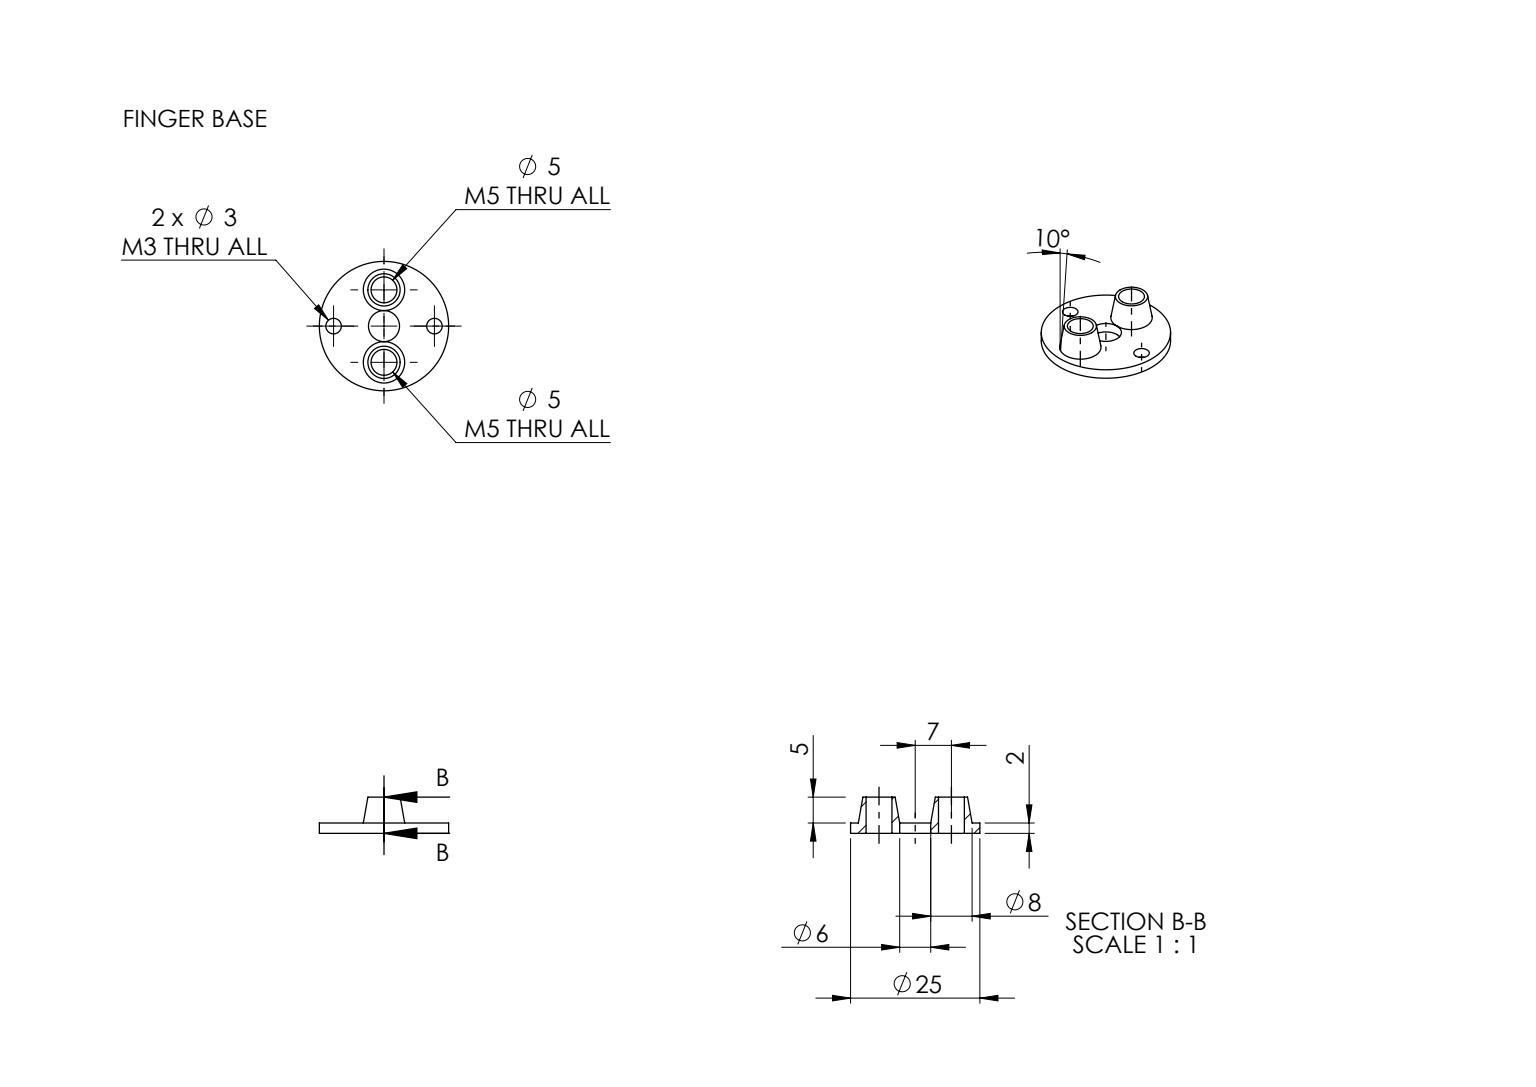
ISO-10303-21;
HEADER;
FILE_DESCRIPTION (('STEP AP214'),
    '1' );
FILE_NAME ('finger base.step',
    '2026-10-04T10:31:01',
    ( '' ),
    ( '' ),
    'SwSTEP 2.0',
    'SolidWorks 2026',
    '' );
FILE_SCHEMA (( 'AUTOMOTIVE_DESIGN' ));
ENDSEC;

DATA;
#8=ORIENTED_EDGE ( 'NONE', *, *, #4476, .T. ) ;
#18=LINE ( 'NONE', #14576, #2348 ) ;
#22=CARTESIAN_POINT ( 'NONE',  ( -3.061616997868391523E-16, 189.0000000000000000, -7.000000000000000000 ) ) ;
#42=EDGE_CURVE ( 'NONE', #14222, #12950, #1605, .T. ) ;
#113=EDGE_CURVE ( 'NONE', #5247, #7816, #14877, .T. ) ;
#127=CARTESIAN_POINT ( 'NONE',  ( 0.000000000000000000, 184.0000000000000000, 0.000000000000000000 ) ) ;
#147=DIRECTION ( 'NONE',  ( -1.000000000000000000, 0.000000000000000000, 0.000000000000000000 ) ) ;
#166=PRODUCT ( 'finger base', 'finger base', '', ( #15382 ) ) ;
#182=DIRECTION ( 'NONE',  ( -0.1736481776669306920, -0.9848077530122080203, 0.000000000000000000 ) ) ;
#199=CIRCLE ( 'NONE', #5549, 2.499999999999999556 ) ;
#215=SURFACE_SIDE_STYLE ('',( #11110 ) ) ;
#260=VERTEX_POINT ( 'NONE', #5788 ) ;
#261=ORIENTED_EDGE ( 'NONE', *, *, #6781, .F. ) ;
#280=DIRECTION ( 'NONE',  ( -6.123233995736766036E-17, 1.000000000000000000, 0.000000000000000000 ) ) ;
#285=AXIS2_PLACEMENT_3D ( 'NONE', #127, #3629, #8659 ) ;
#315=ORIENTED_EDGE ( 'NONE', *, *, #1912, .F. ) ;
#323=SURFACE_STYLE_FILL_AREA ( #10269 ) ;
#424=AXIS2_PLACEMENT_3D ( 'NONE', #6276, #8742, #11195 ) ;
#466=CARTESIAN_POINT ( 'NONE',  ( 0.000000000000000000, 184.0000000000000000, 0.000000000000000000 ) ) ;
#476=DIRECTION ( 'NONE',  ( 0.000000000000000000, 0.000000000000000000, 1.000000000000000000 ) ) ;
#481=DIRECTION ( 'NONE',  ( -6.123233995736766036E-17, 1.000000000000000000, 0.000000000000000000 ) ) ;
#509=ORIENTED_EDGE ( 'NONE', *, *, #12250, .F. ) ;
#550=ADVANCED_FACE ( 'NONE', ( #2271 ), #7141, .T. ) ;
#552=DIRECTION ( 'NONE',  ( -6.123233995736766036E-17, 1.000000000000000000, 0.000000000000000000 ) ) ;
#561=DIRECTION ( 'NONE',  ( -0.000000000000000000, 1.000000000000000000, -0.000000000000000000 ) ) ;
#562=PLANE ( 'NONE',  #12276 ) ;
#622=ORIENTED_EDGE ( 'NONE', *, *, #10760, .T. ) ;
#633=DIRECTION ( 'NONE',  ( 0.000000000000000000, 0.000000000000000000, 1.000000000000000000 ) ) ;
#640=EDGE_LOOP ( 'NONE', ( #3910, #10945 ) ) ;
#650=CARTESIAN_POINT ( 'NONE',  ( -9.148167235839370302E-31, 189.0000000000000000, 4.500000000000000888 ) ) ;
#658=ORIENTED_EDGE ( 'NONE', *, *, #14770, .T. ) ;
#700=CONICAL_SURFACE ( 'NONE', #15707, 4.000000000000001776, 0.1745329251994333364 ) ;
#702=CIRCLE ( 'NONE', #11125, 12.49999999999999822 ) ;
#742=CIRCLE ( 'NONE', #2268, 1.499999999999999556 ) ;
#803=AXIS2_PLACEMENT_3D ( 'NONE', #2594, #12294, #1393 ) ;
#842=EDGE_CURVE ( 'NONE', #7816, #5381, #5978, .T. ) ;
#847=ORIENTED_EDGE ( 'NONE', *, *, #12750, .T. ) ;
#877=EDGE_CURVE ( 'NONE', #5381, #5666, #1680, .T. ) ;
#896=CARTESIAN_POINT ( 'NONE',  ( -4.000000000000002665, 184.0000000000000000, -7.000000000000000000 ) ) ;
#918=AXIS2_PLACEMENT_3D ( 'NONE', #466, #15034, #6295 ) ;
#934=DIRECTION ( 'NONE',  ( -6.123233995736766036E-17, 1.000000000000000000, 0.000000000000000000 ) ) ;
#955=DIRECTION ( 'NONE',  ( 1.000000000000000000, 6.123233995736766036E-17, 0.000000000000000000 ) ) ;
#990=CARTESIAN_POINT ( 'NONE',  ( 0.000000000000000000, 184.0000000000000000, 2.999999999999998224 ) ) ;
#999=AXIS2_PLACEMENT_3D ( 'NONE', #13899, #6603, #9146 ) ;
#1019=ORIENTED_EDGE ( 'NONE', *, *, #5618, .F. ) ;
#1037=ADVANCED_FACE ( 'NONE', ( #2861 ), #6531, .F. ) ;
#1043=EDGE_CURVE ( 'NONE', #4972, #8636, #4494, .T. ) ;
#1061=VERTEX_POINT ( 'NONE', #12635 ) ;
#1081=EDGE_LOOP ( 'NONE', ( #14981, #4075, #14585, #5983 ) ) ;
#1165=( NAMED_UNIT ( * ) PLANE_ANGLE_UNIT ( ) SI_UNIT ( $, .RADIAN. ) );
#1203=AXIS2_PLACEMENT_3D ( 'NONE', #11068, #5988, #10992 ) ;
#1257=ADVANCED_FACE ( 'NONE', ( #11272 ), #7034, .T. ) ;
#1260=CARTESIAN_POINT ( 'NONE',  ( 1.530808498934191324E-15, 184.0000000000000000, 12.49999999999999822 ) ) ;
#1347=CARTESIAN_POINT ( 'NONE',  ( 9.750000000000003553, 184.0000000000000000, 1.020968533498575461E-13 ) ) ;
#1355=EDGE_CURVE ( 'NONE', #5666, #5381, #15411, .T. ) ;
#1370=ORIENTED_EDGE ( 'NONE', *, *, #3477, .F. ) ;
#1388=CARTESIAN_POINT ( 'NONE',  ( -3.061616997868391523E-16, 182.0000000000000000, 7.000000000000000000 ) ) ;
#1393=DIRECTION ( 'NONE',  ( -1.000000000000000000, 0.000000000000000000, 0.000000000000000000 ) ) ;
#1418=VECTOR ( 'NONE', #14560, 1000.000000000000000 ) ;
#1427=ADVANCED_FACE ( 'NONE', ( #12848 ), #1951, .F. ) ;
#1463=VECTOR ( 'NONE', #561, 1000.000000000000000 ) ;
#1473=DIRECTION ( 'NONE',  ( 0.000000000000000000, 0.000000000000000000, 1.000000000000000000 ) ) ;
#1488=ORIENTED_EDGE ( 'NONE', *, *, #10760, .F. ) ;
#1491=CARTESIAN_POINT ( 'NONE',  ( -3.061616997868386099E-16, 189.0000000000000000, 7.000000000000000000 ) ) ;
#1589=FILL_AREA_STYLE_COLOUR ( '', #14448 ) ;
#1605=LINE ( 'NONE', #2653, #14618 ) ;
#1609=CONICAL_SURFACE ( 'NONE', #3645, 4.000000000000002665, 0.1745329251994333364 ) ;
#1651=DIRECTION ( 'NONE',  ( 1.000000000000000000, 0.000000000000000000, 0.000000000000000000 ) ) ;
#1658=DIRECTION ( 'NONE',  ( -0.000000000000000000, 1.000000000000000000, -0.000000000000000000 ) ) ;
#1679=EDGE_LOOP ( 'NONE', ( #2885, #13212 ) ) ;
#1680=CIRCLE ( 'NONE', #12608, 1.499999999999999556 ) ;
#1701=CARTESIAN_POINT ( 'NONE',  ( 3.118365096457674568, 189.0000000000000000, -7.000000000000000888 ) ) ;
#1715=CARTESIAN_POINT ( 'NONE',  ( -9.750000000000003553, 184.0000000000000000, -3.401296724241641415E-14 ) ) ;
#1721=AXIS2_PLACEMENT_3D ( 'NONE', #13992, #15511, #9156 ) ;
#1725=VECTOR ( 'NONE', #7804, 1000.000000000000000 ) ;
#1726=DIRECTION ( 'NONE',  ( -6.123233995736766036E-17, 1.000000000000000000, 0.000000000000000000 ) ) ;
#1736=AXIS2_PLACEMENT_3D ( 'NONE', #2792, #8928, #476 ) ;
#1743=CYLINDRICAL_SURFACE ( 'NONE', #1746, 2.499999999999999556 ) ;
#1746=AXIS2_PLACEMENT_3D ( 'NONE', #5265, #10342, #12567 ) ;
#1809=CARTESIAN_POINT ( 'NONE',  ( -3.061616997868391523E-16, 189.0000000000000000, -7.000000000000000000 ) ) ;
#1833=ORIENTED_EDGE ( 'NONE', *, *, #2892, .T. ) ;
#1898=DIRECTION ( 'NONE',  ( -1.000000000000000000, 0.000000000000000000, 0.000000000000000000 ) ) ;
#1908=AXIS2_PLACEMENT_3D ( 'NONE', #3067, #5542, #5467 ) ;
#1912=EDGE_CURVE ( 'NONE', #2813, #6711, #6038, .T. ) ;
#1931=CYLINDRICAL_SURFACE ( 'NONE', #4961, 1.499999999999999556 ) ;
#1951=CYLINDRICAL_SURFACE ( 'NONE', #5267, 1.499999999999999556 ) ;
#1981=DIRECTION ( 'NONE',  ( 0.000000000000000000, 0.000000000000000000, 1.000000000000000000 ) ) ;
#1997=CARTESIAN_POINT ( 'NONE',  ( 9.750000000000003553, 184.0000000000000000, 1.020968533498575461E-13 ) ) ;
#2021=CYLINDRICAL_SURFACE ( 'NONE', #1908, 12.49999999999999822 ) ;
#2054=VERTEX_POINT ( 'NONE', #13437 ) ;
#2057=CYLINDRICAL_SURFACE ( 'NONE', #5024, 2.499999999999999556 ) ;
#2067=FACE_BOUND ( 'NONE', #14789, .T. ) ;
#2071=AXIS2_PLACEMENT_3D ( 'NONE', #15163, #5148, #1473 ) ;
#2095=ORIENTED_EDGE ( 'NONE', *, *, #3370, .F. ) ;
#2105=EDGE_CURVE ( 'NONE', #6711, #2813, #8603, .T. ) ;
#2110=LINE ( 'NONE', #13086, #8853 ) ;
#2196=( NAMED_UNIT ( * ) SI_UNIT ( $, .STERADIAN. ) SOLID_ANGLE_UNIT ( ) );
#2211=DIRECTION ( 'NONE',  ( 0.000000000000000000, 0.000000000000000000, 1.000000000000000000 ) ) ;
#2214=CARTESIAN_POINT ( 'NONE',  ( 9.750000000000003553, 182.0000000000000000, 1.020968533498575461E-13 ) ) ;
#2240=EDGE_CURVE ( 'NONE', #10282, #13993, #5485, .T. ) ;
#2247=DIRECTION ( 'NONE',  ( 6.123233995736766036E-17, -1.000000000000000000, -0.000000000000000000 ) ) ;
#2254=ORIENTED_EDGE ( 'NONE', *, *, #7655, .F. ) ;
#2268=AXIS2_PLACEMENT_3D ( 'NONE', #14846, #11337, #6504 ) ;
#2271=FACE_OUTER_BOUND ( 'NONE', #6770, .T. ) ;
#2279=FILL_AREA_STYLE ('',( #13180 ) ) ;
#2295=DIRECTION ( 'NONE',  ( 6.123233995736766036E-17, -1.000000000000000000, -0.000000000000000000 ) ) ;
#2317=FACE_OUTER_BOUND ( 'NONE', #1081, .T. ) ;
#2324=ORIENTED_EDGE ( 'NONE', *, *, #11630, .T. ) ;
#2348=VECTOR ( 'NONE', #3673, 1000.000000000000000 ) ;
#2373=AXIS2_PLACEMENT_3D ( 'NONE', #7244, #4937, #9866 ) ;
#2455=ORIENTED_EDGE ( 'NONE', *, *, #4255, .T. ) ;
#2484=AXIS2_PLACEMENT_3D ( 'NONE', #13916, #481, #8852 ) ;
#2497=AXIS2_PLACEMENT_3D ( 'NONE', #1809, #12555, #7869 ) ;
#2540=CARTESIAN_POINT ( 'NONE',  ( 9.750000000000003553, 182.0000000000000000, -1.499999999999897415 ) ) ;
#2579=CARTESIAN_POINT ( 'NONE',  ( 0.000000000000000000, 182.0000000000000000, 0.000000000000000000 ) ) ;
#2582=PRODUCT_DEFINITION_SHAPE ( 'NONE', 'NONE',  #3028 ) ;
#2594=CARTESIAN_POINT ( 'NONE',  ( -3.061616997868386099E-16, 189.0000000000000000, -7.000000000000000000 ) ) ;
#2615=AXIS2_PLACEMENT_3D ( 'NONE', #10996, #9813, #12262 ) ;
#2639=LINE ( 'NONE', #12495, #7435 ) ;
#2653=CARTESIAN_POINT ( 'NONE',  ( -4.000000000000002665, 184.0000000000000000, -7.000000000000000000 ) ) ;
#2670=CARTESIAN_POINT ( 'NONE',  ( 1.530808498934191324E-15, 182.0000000000000000, 12.49999999999999822 ) ) ;
#2682=CARTESIAN_POINT ( 'NONE',  ( 0.000000000000000000, 184.0000000000000000, -12.49999999999999822 ) ) ;
#2685=CARTESIAN_POINT ( 'NONE',  ( 9.750000000000003553, 184.0000000000000000, 1.020968533498575461E-13 ) ) ;
#2694=EDGE_CURVE ( 'NONE', #10558, #13993, #8074, .T. ) ;
#2706=ORIENTED_EDGE ( 'NONE', *, *, #113, .F. ) ;
#2720=FACE_OUTER_BOUND ( 'NONE', #14878, .T. ) ;
#2740=EDGE_CURVE ( 'NONE', #10533, #8352, #14159, .T. ) ;
#2790=ORIENTED_EDGE ( 'NONE', *, *, #2740, .T. ) ;
#2791=FACE_BOUND ( 'NONE', #14523, .T. ) ;
#2792=CARTESIAN_POINT ( 'NONE',  ( -9.750000000000003553, 182.0000000000000000, -3.401296724241641415E-14 ) ) ;
#2813=VERTEX_POINT ( 'NONE', #5350 ) ;
#2861=FACE_OUTER_BOUND ( 'NONE', #11217, .T. ) ;
#2877=EDGE_CURVE ( 'NONE', #13893, #6615, #5812, .T. ) ;
#2885=ORIENTED_EDGE ( 'NONE', *, *, #13327, .F. ) ;
#2892=EDGE_CURVE ( 'NONE', #7816, #5247, #6563, .T. ) ;
#2908=CARTESIAN_POINT ( 'NONE',  ( 0.000000000000000000, 184.0000000000000000, -7.000000000000000000 ) ) ;
#2935=ADVANCED_FACE ( 'NONE', ( #14071 ), #2057, .F. ) ;
#2941=DIRECTION ( 'NONE',  ( 0.000000000000000000, 0.000000000000000000, 1.000000000000000000 ) ) ;
#2948=FACE_OUTER_BOUND ( 'NONE', #13927, .T. ) ;
#2954=CARTESIAN_POINT ( 'NONE',  ( 3.118365096457673680, 189.0000000000000000, 7.000000000000000000 ) ) ;
#2961=ORIENTED_EDGE ( 'NONE', *, *, #1355, .T. ) ;
#2967=ORIENTED_EDGE ( 'NONE', *, *, #3402, .F. ) ;
#2984=EDGE_CURVE ( 'NONE', #9629, #13232, #9852, .T. ) ;
#3010=FACE_OUTER_BOUND ( 'NONE', #11955, .T. ) ;
#3018=LINE ( 'NONE', #12481, #15604 ) ;
#3028=PRODUCT_DEFINITION ( 'UNKNOWN', '', #12132, #10242 ) ;
#3033=CARTESIAN_POINT ( 'NONE',  ( -3.061616997868391523E-16, 182.0000000000000000, 7.000000000000000000 ) ) ;
#3067=CARTESIAN_POINT ( 'NONE',  ( 0.000000000000000000, 184.0000000000000000, 0.000000000000000000 ) ) ;
#3101=DIRECTION ( 'NONE',  ( 0.000000000000000000, 0.000000000000000000, -1.000000000000000000 ) ) ;
#3111=DIRECTION ( 'NONE',  ( 0.000000000000000000, -1.000000000000000000, 0.000000000000000000 ) ) ;
#3175=EDGE_LOOP ( 'NONE', ( #5886, #5946, #4607, #11234, #14651, #4654, #3423, #5027 ) ) ;
#3296=CIRCLE ( 'NONE', #5081, 4.000000000000002665 ) ;
#3370=EDGE_CURVE ( 'NONE', #11100, #2054, #199, .T. ) ;
#3402=EDGE_CURVE ( 'NONE', #5247, #5666, #6779, .T. ) ;
#3423=ORIENTED_EDGE ( 'NONE', *, *, #10805, .F. ) ;
#3449=CARTESIAN_POINT ( 'NONE',  ( 1.530808498934191324E-15, 184.0000000000000000, 12.49999999999999822 ) ) ;
#3461=EDGE_CURVE ( 'NONE', #10282, #12193, #7572, .T. ) ;
#3477=EDGE_CURVE ( 'NONE', #6711, #260, #8935, .T. ) ;
#3478=CARTESIAN_POINT ( 'NONE',  ( 0.000000000000000000, 184.0000000000000000, -2.999999999999997335 ) ) ;
#3487=ORIENTED_EDGE ( 'NONE', *, *, #3658, .F. ) ;
#3491=CARTESIAN_POINT ( 'NONE',  ( 0.000000000000000000, 184.0000000000000000, -7.000000000000000000 ) ) ;
#3504=EDGE_CURVE ( 'NONE', #13993, #10558, #702, .T. ) ;
#3505=EDGE_LOOP ( 'NONE', ( #3953, #12586 ) ) ;
#3523=CIRCLE ( 'NONE', #4807, 3.118365096457675012 ) ;
#3629=DIRECTION ( 'NONE',  ( 0.000000000000000000, -1.000000000000000000, 0.000000000000000000 ) ) ;
#3645=AXIS2_PLACEMENT_3D ( 'NONE', #3491, #2295, #147 ) ;
#3658=EDGE_CURVE ( 'NONE', #12135, #14543, #7170, .T. ) ;
#3662=ORIENTED_EDGE ( 'NONE', *, *, #14129, .T. ) ;
#3672=AXIS2_PLACEMENT_3D ( 'NONE', #5276, #3111, #9168 ) ;
#3673=DIRECTION ( 'NONE',  ( 0.000000000000000000, -1.000000000000000000, 0.000000000000000000 ) ) ;
#3684=CLOSED_SHELL ( 'NONE', ( #14930, #14667, #12649, #1427, #8535, #1257, #1037, #550, #9243, #10383, #8764, #14579, #14863, #12972, #10318, #10276, #12271, #15514, #2935, #6306 ) ) ;
#3718=ORIENTED_EDGE ( 'NONE', *, *, #1355, .F. ) ;
#3732=DIRECTION ( 'NONE',  ( 0.000000000000000000, -1.000000000000000000, 0.000000000000000000 ) ) ;
#3735=DIRECTION ( 'NONE',  ( -0.000000000000000000, 1.000000000000000000, -0.000000000000000000 ) ) ;
#3786=EDGE_CURVE ( 'NONE', #12193, #10282, #15197, .T. ) ;
#3875=ORIENTED_EDGE ( 'NONE', *, *, #3786, .T. ) ;
#3889=ORIENTED_EDGE ( 'NONE', *, *, #113, .T. ) ;
#3896=EDGE_LOOP ( 'NONE', ( #8438, #14161, #4789, #13602 ) ) ;
#3901=AXIS2_PLACEMENT_3D ( 'NONE', #10495, #934, #14062 ) ;
#3910=ORIENTED_EDGE ( 'NONE', *, *, #12092, .T. ) ;
#3953=ORIENTED_EDGE ( 'NONE', *, *, #2105, .T. ) ;
#3974=EDGE_LOOP ( 'NONE', ( #9767, #9319 ) ) ;
#3988=ORIENTED_EDGE ( 'NONE', *, *, #2984, .T. ) ;
#4042=( GEOMETRIC_REPRESENTATION_CONTEXT ( 3 ) GLOBAL_UNCERTAINTY_ASSIGNED_CONTEXT ( ( #6173 ) ) GLOBAL_UNIT_ASSIGNED_CONTEXT ( ( #14055, #8020, #2196 ) ) REPRESENTATION_CONTEXT ( 'NONE', 'WORKASPACE' ) );
#4055=EDGE_CURVE ( 'NONE', #12288, #4510, #9356, .T. ) ;
#4057=CARTESIAN_POINT ( 'NONE',  ( -3.061616997868386099E-16, 189.0000000000000000, -7.000000000000000000 ) ) ;
#4065=CARTESIAN_POINT ( 'NONE',  ( 9.750000000000003553, 184.0000000000000000, -1.499999999999897415 ) ) ;
#4075=ORIENTED_EDGE ( 'NONE', *, *, #2877, .T. ) ;
#4078=EDGE_LOOP ( 'NONE', ( #1488, #2095, #14503, #3988 ) ) ;
#4142=DIRECTION ( 'NONE',  ( 0.000000000000000000, 0.000000000000000000, -1.000000000000000000 ) ) ;
#4158=DIRECTION ( 'NONE',  ( 0.000000000000000000, 0.000000000000000000, 1.000000000000000000 ) ) ;
#4166=CARTESIAN_POINT ( 'NONE',  ( 0.000000000000000000, 184.0000000000000000, 0.000000000000000000 ) ) ;
#4200=AXIS2_PLACEMENT_3D ( 'NONE', #7400, #9870, #6218 ) ;
#4229=ORIENTED_EDGE ( 'NONE', *, *, #3504, .T. ) ;
#4230=EDGE_LOOP ( 'NONE', ( #509, #7952, #10338, #2455 ) ) ;
#4231=AXIS2_PLACEMENT_3D ( 'NONE', #12227, #6201, #11038 ) ;
#4255=EDGE_CURVE ( 'NONE', #4510, #12288, #14712, .T. ) ;
#4295=SURFACE_SIDE_STYLE ('',( #323 ) ) ;
#4311=ORIENTED_EDGE ( 'NONE', *, *, #12250, .T. ) ;
#4406=DIRECTION ( 'NONE',  ( 0.000000000000000000, 0.000000000000000000, -1.000000000000000000 ) ) ;
#4444=DIRECTION ( 'NONE',  ( -0.000000000000000000, 1.000000000000000000, -0.000000000000000000 ) ) ;
#4469=DIRECTION ( 'NONE',  ( 0.000000000000000000, 0.000000000000000000, 1.000000000000000000 ) ) ;
#4476=EDGE_CURVE ( 'NONE', #9576, #10284, #742, .T. ) ;
#4488=ORIENTED_EDGE ( 'NONE', *, *, #2240, .T. ) ;
#4494=CIRCLE ( 'NONE', #5763, 2.499999999999999556 ) ;
#4510=VERTEX_POINT ( 'NONE', #5226 ) ;
#4549=ORIENTED_EDGE ( 'NONE', *, *, #877, .F. ) ;
#4551=AXIS2_PLACEMENT_3D ( 'NONE', #12645, #10268, #3101 ) ;
#4555=EDGE_CURVE ( 'NONE', #12950, #12135, #3296, .T. ) ;
#4607=ORIENTED_EDGE ( 'NONE', *, *, #7801, .F. ) ;
#4610=CARTESIAN_POINT ( 'NONE',  ( -8.666684749742561339E-31, 189.0000000000000000, 4.500000000000000888 ) ) ;
#4654=ORIENTED_EDGE ( 'NONE', *, *, #14129, .F. ) ;
#4777=DIRECTION ( 'NONE',  ( 0.000000000000000000, 0.000000000000000000, 1.000000000000000000 ) ) ;
#4781=DIRECTION ( 'NONE',  ( 0.000000000000000000, 0.000000000000000000, -1.000000000000000000 ) ) ;
#4789=ORIENTED_EDGE ( 'NONE', *, *, #13716, .T. ) ;
#4793=AXIS2_PLACEMENT_3D ( 'NONE', #11299, #8617, #12411 ) ;
#4807=AXIS2_PLACEMENT_3D ( 'NONE', #4057, #552, #1898 ) ;
#4812=DIRECTION ( 'NONE',  ( -6.123233995736766036E-17, 1.000000000000000000, 0.000000000000000000 ) ) ;
#4820=DIRECTION ( 'NONE',  ( -0.1736481776669306920, -0.9848077530122080203, 2.126576849575776229E-17 ) ) ;
#4859=CARTESIAN_POINT ( 'NONE',  ( -3.061616997868391523E-16, 189.0000000000000000, 7.000000000000000000 ) ) ;
#4937=DIRECTION ( 'NONE',  ( -6.123233995736766036E-17, 1.000000000000000000, 0.000000000000000000 ) ) ;
#4943=MANIFOLD_SOLID_BREP ( 'AdvancedHole3', #3684 ) ;
#4961=AXIS2_PLACEMENT_3D ( 'NONE', #8228, #15308, #13063 ) ;
#4965=EDGE_CURVE ( 'NONE', #1061, #6866, #9367, .T. ) ;
#4969=ORIENTED_EDGE ( 'NONE', *, *, #3477, .T. ) ;
#4972=VERTEX_POINT ( 'NONE', #5346 ) ;
#5024=AXIS2_PLACEMENT_3D ( 'NONE', #13036, #6933, #10737 ) ;
#5027=ORIENTED_EDGE ( 'NONE', *, *, #2740, .F. ) ;
#5032=CARTESIAN_POINT ( 'NONE',  ( -9.750000000000003553, 182.0000000000000000, 1.499999999999965583 ) ) ;
#5044=ORIENTED_EDGE ( 'NONE', *, *, #10805, .T. ) ;
#5081=AXIS2_PLACEMENT_3D ( 'NONE', #2908, #280, #5144 ) ;
#5139=EDGE_CURVE ( 'NONE', #8636, #4972, #14462, .T. ) ;
#5144=DIRECTION ( 'NONE',  ( -1.000000000000000000, 0.000000000000000000, 0.000000000000000000 ) ) ;
#5148=DIRECTION ( 'NONE',  ( -0.000000000000000000, 1.000000000000000000, -0.000000000000000000 ) ) ;
#5226=CARTESIAN_POINT ( 'NONE',  ( -3.061616997868391523E-16, 189.0000000000000000, -4.500000000000000888 ) ) ;
#5242=CYLINDRICAL_SURFACE ( 'NONE', #6310, 1.499999999999999556 ) ;
#5247=VERTEX_POINT ( 'NONE', #2540 ) ;
#5265=CARTESIAN_POINT ( 'NONE',  ( -3.061616997868391523E-16, 189.0000000000000000, -7.000000000000000000 ) ) ;
#5267=AXIS2_PLACEMENT_3D ( 'NONE', #1715, #14198, #11426 ) ;
#5276=CARTESIAN_POINT ( 'NONE',  ( 0.000000000000000000, 182.0000000000000000, 0.000000000000000000 ) ) ;
#5346=CARTESIAN_POINT ( 'NONE',  ( -3.061616997868391523E-16, 182.0000000000000000, -4.500000000000000888 ) ) ;
#5350=CARTESIAN_POINT ( 'NONE',  ( -3.118365096457674568, 189.0000000000000000, 7.000000000000000888 ) ) ;
#5361=EDGE_LOOP ( 'NONE', ( #315, #15554, #5044, #1370 ) ) ;
#5381=VERTEX_POINT ( 'NONE', #8015 ) ;
#5421=AXIS2_PLACEMENT_3D ( 'NONE', #6879, #10450, #4406 ) ;
#5430=CARTESIAN_POINT ( 'NONE',  ( 0.000000000000000000, 184.0000000000000000, 0.000000000000000000 ) ) ;
#5467=DIRECTION ( 'NONE',  ( 0.000000000000000000, 0.000000000000000000, -1.000000000000000000 ) ) ;
#5485=LINE ( 'NONE', #3449, #14411 ) ;
#5497=EDGE_CURVE ( 'NONE', #11100, #9629, #10636, .T. ) ;
#5506=DIRECTION ( 'NONE',  ( 0.000000000000000000, -1.000000000000000000, 0.000000000000000000 ) ) ;
#5513=EDGE_LOOP ( 'NONE', ( #13468, #13148 ) ) ;
#5530=LINE ( 'NONE', #14028, #7742 ) ;
#5542=DIRECTION ( 'NONE',  ( 0.000000000000000000, -1.000000000000000000, 0.000000000000000000 ) ) ;
#5549=AXIS2_PLACEMENT_3D ( 'NONE', #3033, #14001, #633 ) ;
#5618=EDGE_CURVE ( 'NONE', #10533, #12135, #7159, .T. ) ;
#5666=VERTEX_POINT ( 'NONE', #12531 ) ;
#5745=ORIENTED_EDGE ( 'NONE', *, *, #3658, .T. ) ;
#5763=AXIS2_PLACEMENT_3D ( 'NONE', #9000, #13828, #2941 ) ;
#5788=CARTESIAN_POINT ( 'NONE',  ( 4.000000000000001776, 184.0000000000000000, 7.000000000000000000 ) ) ;
#5812=LINE ( 'NONE', #10577, #11114 ) ;
#5861=DIRECTION ( 'NONE',  ( -0.000000000000000000, 1.000000000000000000, -0.000000000000000000 ) ) ;
#5877=APPLICATION_CONTEXT ( 'automotive_design' ) ;
#5886=ORIENTED_EDGE ( 'NONE', *, *, #5618, .T. ) ;
#5887=CARTESIAN_POINT ( 'NONE',  ( -3.061616997868391523E-16, 182.0000000000000000, -7.000000000000000000 ) ) ;
#5946=ORIENTED_EDGE ( 'NONE', *, *, #4555, .F. ) ;
#5978=LINE ( 'NONE', #13362, #1418 ) ;
#5983=ORIENTED_EDGE ( 'NONE', *, *, #42, .F. ) ;
#5988=DIRECTION ( 'NONE',  ( 0.000000000000000000, -1.000000000000000000, 0.000000000000000000 ) ) ;
#6003=DIRECTION ( 'NONE',  ( 1.000000000000000000, 0.000000000000000000, 0.000000000000000000 ) ) ;
#6034=( LENGTH_UNIT ( ) NAMED_UNIT ( * ) SI_UNIT ( .MILLI., .METRE. ) );
#6038=CIRCLE ( 'NONE', #13391, 3.118365096457674124 ) ;
#6067=ORIENTED_EDGE ( 'NONE', *, *, #4055, .T. ) ;
#6092=COLOUR_RGB ( '', 0.66274510, 0.83137255, 0.94901961) ;
#6105=MECHANICAL_DESIGN_GEOMETRIC_PRESENTATION_REPRESENTATION('',(#9157),#6368);
#6107=CARTESIAN_POINT ( 'NONE',  ( -9.750000000000003553, 184.0000000000000000, 1.499999999999965583 ) ) ;
#6173=UNCERTAINTY_MEASURE_WITH_UNIT (LENGTH_MEASURE( 1.000000000000000082E-05 ), #14055, 'distance_accuracy_value', 'NONE');
#6189=DIRECTION ( 'NONE',  ( 0.000000000000000000, 0.000000000000000000, -1.000000000000000000 ) ) ;
#6201=DIRECTION ( 'NONE',  ( -0.000000000000000000, 1.000000000000000000, -0.000000000000000000 ) ) ;
#6218=DIRECTION ( 'NONE',  ( 1.000000000000000000, 0.000000000000000000, 0.000000000000000000 ) ) ;
#6263=DIRECTION ( 'NONE',  ( -0.000000000000000000, 1.000000000000000000, -0.000000000000000000 ) ) ;
#6271=( NAMED_UNIT ( * ) SI_UNIT ( $, .STERADIAN. ) SOLID_ANGLE_UNIT ( ) );
#6276=CARTESIAN_POINT ( 'NONE',  ( 0.000000000000000000, 184.0000000000000000, 7.000000000000000000 ) ) ;
#6295=DIRECTION ( 'NONE',  ( 0.000000000000000000, 0.000000000000000000, -1.000000000000000000 ) ) ;
#6297=EDGE_CURVE ( 'NONE', #14222, #13893, #14797, .T. ) ;
#6302=ORIENTED_EDGE ( 'NONE', *, *, #10587, .F. ) ;
#6303=AXIS2_PLACEMENT_3D ( 'NONE', #1491, #1726, #13819 ) ;
#6306=ADVANCED_FACE ( 'NONE', ( #6432 ), #13959, .F. ) ;
#6310=AXIS2_PLACEMENT_3D ( 'NONE', #2685, #13502, #8670 ) ;
#6314=VECTOR ( 'NONE', #9240, 1000.000000000000000 ) ;
#6357=DIRECTION ( 'NONE',  ( -6.123233995736766036E-17, 1.000000000000000000, 0.000000000000000000 ) ) ;
#6368=( GEOMETRIC_REPRESENTATION_CONTEXT ( 3 ) GLOBAL_UNCERTAINTY_ASSIGNED_CONTEXT ( ( #14429 ) ) GLOBAL_UNIT_ASSIGNED_CONTEXT ( ( #6034, #1165, #6271 ) ) REPRESENTATION_CONTEXT ( 'NONE', 'WORKASPACE' ) );
#6432=FACE_OUTER_BOUND ( 'NONE', #4078, .T. ) ;
#6504=DIRECTION ( 'NONE',  ( 0.000000000000000000, 0.000000000000000000, 1.000000000000000000 ) ) ;
#6531=CYLINDRICAL_SURFACE ( 'NONE', #918, 3.000000000000000888 ) ;
#6535=ORIENTED_EDGE ( 'NONE', *, *, #8176, .F. ) ;
#6539=FACE_OUTER_BOUND ( 'NONE', #13454, .T. ) ;
#6540=PRESENTATION_STYLE_ASSIGNMENT (( #6620 ) ) ;
#6563=CIRCLE ( 'NONE', #10601, 1.499999999999999556 ) ;
#6603=DIRECTION ( 'NONE',  ( -0.000000000000000000, 1.000000000000000000, -0.000000000000000000 ) ) ;
#6605=AXIS2_PLACEMENT_3D ( 'NONE', #5887, #10734, #2211 ) ;
#6615=VERTEX_POINT ( 'NONE', #9587 ) ;
#6620=SURFACE_STYLE_USAGE ( .BOTH. , #4295 ) ;
#6655=ORIENTED_EDGE ( 'NONE', *, *, #3461, .T. ) ;
#6680=CARTESIAN_POINT ( 'NONE',  ( 0.000000000000000000, 0.000000000000000000, 0.000000000000000000 ) ) ;
#6696=( NAMED_UNIT ( * ) SI_UNIT ( $, .STERADIAN. ) SOLID_ANGLE_UNIT ( ) );
#6711=VERTEX_POINT ( 'NONE', #2954 ) ;
#6770=EDGE_LOOP ( 'NONE', ( #3875, #4488, #10302, #261 ) ) ;
#6775=DIRECTION ( 'NONE',  ( 0.1736481776669307753, -0.9848077530122080203, -2.126576849575776229E-17 ) ) ;
#6779=LINE ( 'NONE', #4065, #1463 ) ;
#6781=EDGE_CURVE ( 'NONE', #12193, #10558, #2639, .T. ) ;
#6790=DIRECTION ( 'NONE',  ( -0.000000000000000000, 1.000000000000000000, -0.000000000000000000 ) ) ;
#6791=CARTESIAN_POINT ( 'NONE',  ( 3.673940397442060854E-16, 182.0000000000000000, 3.000000000000000888 ) ) ;
#6805=CARTESIAN_POINT ( 'NONE',  ( -8.185202263645752375E-31, 189.0000000000000000, -9.500000000000000000 ) ) ;
#6832=VECTOR ( 'NONE', #12213, 1000.000000000000000 ) ;
#6836=AXIS2_PLACEMENT_3D ( 'NONE', #22, #14580, #12031 ) ;
#6855=DIRECTION ( 'NONE',  ( -0.000000000000000000, 1.000000000000000000, -0.000000000000000000 ) ) ;
#6864=ORIENTED_EDGE ( 'NONE', *, *, #842, .F. ) ;
#6866=VERTEX_POINT ( 'NONE', #5032 ) ;
#6879=CARTESIAN_POINT ( 'NONE',  ( 0.000000000000000000, 182.0000000000000000, 0.000000000000000000 ) ) ;
#6924=CARTESIAN_POINT ( 'NONE',  ( -9.750000000000003553, 184.0000000000000000, -1.500000000000033751 ) ) ;
#6933=DIRECTION ( 'NONE',  ( -0.000000000000000000, 1.000000000000000000, -0.000000000000000000 ) ) ;
#6988=DIRECTION ( 'NONE',  ( -0.000000000000000000, 1.000000000000000000, -0.000000000000000000 ) ) ;
#7034=CONICAL_SURFACE ( 'NONE', #424, 4.000000000000001776, 0.1745329251994333364 ) ;
#7126=DIRECTION ( 'NONE',  ( 0.000000000000000000, -1.000000000000000000, 0.000000000000000000 ) ) ;
#7141=CYLINDRICAL_SURFACE ( 'NONE', #7288, 12.49999999999999822 ) ;
#7159=CIRCLE ( 'NONE', #285, 3.000000000000000888 ) ;
#7170=LINE ( 'NONE', #12008, #6314 ) ;
#7244=CARTESIAN_POINT ( 'NONE',  ( -3.061616997868383141E-16, 189.0000000000000000, -7.000000000000000000 ) ) ;
#7245=DIRECTION ( 'NONE',  ( -0.000000000000000000, 1.000000000000000000, -0.000000000000000000 ) ) ;
#7288=AXIS2_PLACEMENT_3D ( 'NONE', #8657, #13254, #6189 ) ;
#7299=EDGE_LOOP ( 'NONE', ( #8558, #6655, #9731, #13452 ) ) ;
#7381=CARTESIAN_POINT ( 'NONE',  ( -3.061616997868391523E-16, 182.0000000000000000, 9.500000000000000000 ) ) ;
#7400=CARTESIAN_POINT ( 'NONE',  ( 0.000000000000000000, 184.0000000000000000, 7.000000000000000000 ) ) ;
#7409=ORIENTED_EDGE ( 'NONE', *, *, #1043, .T. ) ;
#7413=FACE_BOUND ( 'NONE', #5513, .T. ) ;
#7427=ORIENTED_EDGE ( 'NONE', *, *, #4555, .T. ) ;
#7435=VECTOR ( 'NONE', #10120, 1000.000000000000000 ) ;
#7485=EDGE_LOOP ( 'NONE', ( #15397, #847, #8, #8710 ) ) ;
#7488=ORIENTED_EDGE ( 'NONE', *, *, #5139, .T. ) ;
#7502=APPLICATION_CONTEXT ( 'automotive_design' ) ;
#7530=SHAPE_REPRESENTATION_RELATIONSHIP ( 'NONE' , 'NONE' ,  #8978, #12380 ) ;
#7572=CIRCLE ( 'NONE', #14945, 12.49999999999999822 ) ;
#7580=ORIENTED_EDGE ( 'NONE', *, *, #877, .T. ) ;
#7600=DIRECTION ( 'NONE',  ( 0.000000000000000000, 0.000000000000000000, 1.000000000000000000 ) ) ;
#7655=EDGE_CURVE ( 'NONE', #13232, #9629, #14541, .T. ) ;
#7700=EDGE_LOOP ( 'NONE', ( #6302, #14988, #4969, #3662, #2790 ) ) ;
#7703=AXIS2_PLACEMENT_3D ( 'NONE', #15446, #14079, #955 ) ;
#7724=CARTESIAN_POINT ( 'NONE',  ( 0.000000000000000000, 184.0000000000000000, 0.000000000000000000 ) ) ;
#7742=VECTOR ( 'NONE', #15465, 1000.000000000000000 ) ;
#7765=DIRECTION ( 'NONE',  ( -1.000000000000000000, 0.000000000000000000, 0.000000000000000000 ) ) ;
#7796=CYLINDRICAL_SURFACE ( 'NONE', #4551, 3.000000000000000888 ) ;
#7801=EDGE_CURVE ( 'NONE', #6615, #12950, #7940, .T. ) ;
#7804=DIRECTION ( 'NONE',  ( 0.1736481776669307753, -0.9848077530122080203, 0.000000000000000000 ) ) ;
#7816=VERTEX_POINT ( 'NONE', #12534 ) ;
#7832=ORIENTED_EDGE ( 'NONE', *, *, #8351, .T. ) ;
#7864=ORIENTED_EDGE ( 'NONE', *, *, #2694, .T. ) ;
#7869=DIRECTION ( 'NONE',  ( 0.000000000000000000, 0.000000000000000000, 1.000000000000000000 ) ) ;
#7940=CIRCLE ( 'NONE', #13010, 4.000000000000002665 ) ;
#7952=ORIENTED_EDGE ( 'NONE', *, *, #1043, .F. ) ;
#7974=DIRECTION ( 'NONE',  ( -0.000000000000000000, 1.000000000000000000, -0.000000000000000000 ) ) ;
#7983=SHAPE_DEFINITION_REPRESENTATION ( #2582, #8978 ) ;
#7989=ORIENTED_EDGE ( 'NONE', *, *, #42, .T. ) ;
#8004=CIRCLE ( 'NONE', #12313, 1.499999999999999556 ) ;
#8015=CARTESIAN_POINT ( 'NONE',  ( 9.750000000000003553, 184.0000000000000000, 1.500000000000101696 ) ) ;
#8020=( NAMED_UNIT ( * ) PLANE_ANGLE_UNIT ( ) SI_UNIT ( $, .RADIAN. ) );
#8074=CIRCLE ( 'NONE', #1203, 12.49999999999999822 ) ;
#8176=EDGE_CURVE ( 'NONE', #12135, #10533, #12516, .T. ) ;
#8228=CARTESIAN_POINT ( 'NONE',  ( -9.750000000000003553, 184.0000000000000000, -3.401296724241641415E-14 ) ) ;
#8268=CARTESIAN_POINT ( 'NONE',  ( -3.061616997868391523E-16, 189.0000000000000000, 9.500000000000000000 ) ) ;
#8351=EDGE_CURVE ( 'NONE', #14543, #14401, #14034, .T. ) ;
#8352=VERTEX_POINT ( 'NONE', #9259 ) ;
#8367=STYLED_ITEM ( 'NONE', ( #6540 ), #4943 ) ;
#8419=ORIENTED_EDGE ( 'NONE', *, *, #5497, .F. ) ;
#8438=ORIENTED_EDGE ( 'NONE', *, *, #12750, .F. ) ;
#8472=AXIS2_PLACEMENT_3D ( 'NONE', #4166, #10218, #11249 ) ;
#8486=EDGE_CURVE ( 'NONE', #10533, #14401, #18, .T. ) ;
#8535=ADVANCED_FACE ( 'NONE', ( #2317 ), #14284, .T. ) ;
#8540=EDGE_LOOP ( 'NONE', ( #8557, #13620, #7989, #7427, #10674 ) ) ;
#8557=ORIENTED_EDGE ( 'NONE', *, *, #2877, .F. ) ;
#8558=ORIENTED_EDGE ( 'NONE', *, *, #2240, .F. ) ;
#8603=CIRCLE ( 'NONE', #6303, 3.118365096457674124 ) ;
#8609=CARTESIAN_POINT ( 'NONE',  ( 0.000000000000000000, 184.0000000000000000, 0.000000000000000000 ) ) ;
#8612=DIRECTION ( 'NONE',  ( 0.000000000000000000, 0.000000000000000000, 1.000000000000000000 ) ) ;
#8617=DIRECTION ( 'NONE',  ( 0.000000000000000000, -1.000000000000000000, 0.000000000000000000 ) ) ;
#8636=VERTEX_POINT ( 'NONE', #15698 ) ;
#8647=CARTESIAN_POINT ( 'NONE',  ( 4.000000000000001776, 184.0000000000000000, 7.000000000000000000 ) ) ;
#8657=CARTESIAN_POINT ( 'NONE',  ( 0.000000000000000000, 184.0000000000000000, 0.000000000000000000 ) ) ;
#8659=DIRECTION ( 'NONE',  ( 0.000000000000000000, 0.000000000000000000, -1.000000000000000000 ) ) ;
#8662=DIRECTION ( 'NONE',  ( 0.000000000000000000, 0.000000000000000000, 1.000000000000000000 ) ) ;
#8670=DIRECTION ( 'NONE',  ( 0.000000000000000000, 0.000000000000000000, 1.000000000000000000 ) ) ;
#8710=ORIENTED_EDGE ( 'NONE', *, *, #13716, .F. ) ;
#8717=AXIS2_PLACEMENT_3D ( 'NONE', #9775, #14620, #8662 ) ;
#8742=DIRECTION ( 'NONE',  ( 6.123233995736766036E-17, -1.000000000000000000, -0.000000000000000000 ) ) ;
#8764=ADVANCED_FACE ( 'NONE', ( #13844, #9966, #11459, #2720 ), #562, .F. ) ;
#8790=AXIS2_PLACEMENT_3D ( 'NONE', #9322, #6790, #4469 ) ;
#8849=( NAMED_UNIT ( * ) PLANE_ANGLE_UNIT ( ) SI_UNIT ( $, .RADIAN. ) );
#8852=DIRECTION ( 'NONE',  ( 1.000000000000000000, 0.000000000000000000, 0.000000000000000000 ) ) ;
#8853=VECTOR ( 'NONE', #5861, 1000.000000000000000 ) ;
#8866=CIRCLE ( 'NONE', #12663, 2.499999999999999556 ) ;
#8928=DIRECTION ( 'NONE',  ( -0.000000000000000000, 1.000000000000000000, -0.000000000000000000 ) ) ;
#8935=LINE ( 'NONE', #8647, #1725 ) ;
#8946=ORIENTED_EDGE ( 'NONE', *, *, #9439, .F. ) ;
#8978=SHAPE_REPRESENTATION ( 'finger base', ( #14201 ), #4042 ) ;
#9000=CARTESIAN_POINT ( 'NONE',  ( -3.061616997868391523E-16, 182.0000000000000000, -7.000000000000000000 ) ) ;
#9029=CYLINDRICAL_SURFACE ( 'NONE', #10154, 1.499999999999999556 ) ;
#9118=ORIENTED_EDGE ( 'NONE', *, *, #3461, .F. ) ;
#9121=ORIENTED_EDGE ( 'NONE', *, *, #5139, .F. ) ;
#9146=DIRECTION ( 'NONE',  ( 0.000000000000000000, 0.000000000000000000, 1.000000000000000000 ) ) ;
#9156=DIRECTION ( 'NONE',  ( 0.000000000000000000, 0.000000000000000000, 1.000000000000000000 ) ) ;
#9157=STYLED_ITEM ( 'NONE', ( #14698 ), #12380 ) ;
#9168=DIRECTION ( 'NONE',  ( 0.000000000000000000, 0.000000000000000000, -1.000000000000000000 ) ) ;
#9177=FACE_OUTER_BOUND ( 'NONE', #10437, .T. ) ;
#9240=DIRECTION ( 'NONE',  ( 0.000000000000000000, -1.000000000000000000, 0.000000000000000000 ) ) ;
#9243=ADVANCED_FACE ( 'NONE', ( #9245, #2067 ), #11844, .F. ) ;
#9245=FACE_OUTER_BOUND ( 'NONE', #3505, .T. ) ;
#9259=CARTESIAN_POINT ( 'NONE',  ( -4.000000000000001776, 184.0000000000000000, 7.000000000000000888 ) ) ;
#9319=ORIENTED_EDGE ( 'NONE', *, *, #11630, .F. ) ;
#9322=CARTESIAN_POINT ( 'NONE',  ( 9.750000000000003553, 182.0000000000000000, 1.020968533498575461E-13 ) ) ;
#9356=CIRCLE ( 'NONE', #2497, 2.499999999999999556 ) ;
#9367=CIRCLE ( 'NONE', #1736, 1.499999999999999556 ) ;
#9403=ORIENTED_EDGE ( 'NONE', *, *, #8486, .T. ) ;
#9439=EDGE_CURVE ( 'NONE', #4972, #4510, #3018, .T. ) ;
#9576=VERTEX_POINT ( 'NONE', #6924 ) ;
#9587=CARTESIAN_POINT ( 'NONE',  ( 4.000000000000002665, 184.0000000000000000, -7.000000000000000888 ) ) ;
#9620=EDGE_CURVE ( 'NONE', #12135, #6615, #12039, .T. ) ;
#9629=VERTEX_POINT ( 'NONE', #8268 ) ;
#9649=ORIENTED_EDGE ( 'NONE', *, *, #2892, .F. ) ;
#9714=PLANE ( 'NONE',  #2373 ) ;
#9731=ORIENTED_EDGE ( 'NONE', *, *, #6781, .T. ) ;
#9746=EDGE_LOOP ( 'NONE', ( #2706, #15079, #2961, #6864 ) ) ;
#9767=ORIENTED_EDGE ( 'NONE', *, *, #8351, .F. ) ;
#9775=CARTESIAN_POINT ( 'NONE',  ( -3.061616997868391523E-16, 189.0000000000000000, 7.000000000000000000 ) ) ;
#9813=DIRECTION ( 'NONE',  ( 6.123233995736766036E-17, -1.000000000000000000, -0.000000000000000000 ) ) ;
#9852=CIRCLE ( 'NONE', #13897, 2.499999999999999556 ) ;
#9866=DIRECTION ( 'NONE',  ( -1.000000000000000000, -6.123233995736766036E-17, 0.000000000000000000 ) ) ;
#9870=DIRECTION ( 'NONE',  ( -6.123233995736766036E-17, 1.000000000000000000, 0.000000000000000000 ) ) ;
#9942=CARTESIAN_POINT ( 'NONE',  ( -9.750000000000003553, 184.0000000000000000, 1.499999999999965583 ) ) ;
#9966=FACE_BOUND ( 'NONE', #1679, .T. ) ;
#10118=CIRCLE ( 'NONE', #1721, 1.499999999999999556 ) ;
#10120=DIRECTION ( 'NONE',  ( 0.000000000000000000, -1.000000000000000000, 0.000000000000000000 ) ) ;
#10154=AXIS2_PLACEMENT_3D ( 'NONE', #1997, #7974, #4158 ) ;
#10205=ORIENTED_EDGE ( 'NONE', *, *, #4255, .F. ) ;
#10218=DIRECTION ( 'NONE',  ( 0.000000000000000000, -1.000000000000000000, 0.000000000000000000 ) ) ;
#10242=PRODUCT_DEFINITION_CONTEXT ( 'detailed design', #7502, 'design' ) ;
#10268=DIRECTION ( 'NONE',  ( 0.000000000000000000, -1.000000000000000000, 0.000000000000000000 ) ) ;
#10269=FILL_AREA_STYLE ('',( #1589 ) ) ;
#10276=ADVANCED_FACE ( 'NONE', ( #13201, #14552 ), #9714, .T. ) ;
#10282=VERTEX_POINT ( 'NONE', #1260 ) ;
#10284=VERTEX_POINT ( 'NONE', #9942 ) ;
#10302=ORIENTED_EDGE ( 'NONE', *, *, #2694, .F. ) ;
#10318=ADVANCED_FACE ( 'NONE', ( #11049 ), #1609, .T. ) ;
#10338=ORIENTED_EDGE ( 'NONE', *, *, #9439, .T. ) ;
#10342=DIRECTION ( 'NONE',  ( -0.000000000000000000, 1.000000000000000000, -0.000000000000000000 ) ) ;
#10383=ADVANCED_FACE ( 'NONE', ( #10466 ), #2021, .T. ) ;
#10437=EDGE_LOOP ( 'NONE', ( #2967, #9649, #14811, #7580 ) ) ;
#10450=DIRECTION ( 'NONE',  ( 0.000000000000000000, -1.000000000000000000, 0.000000000000000000 ) ) ;
#10456=FACE_OUTER_BOUND ( 'NONE', #3896, .T. ) ;
#10466=FACE_OUTER_BOUND ( 'NONE', #7299, .T. ) ;
#10495=CARTESIAN_POINT ( 'NONE',  ( 0.000000000000000000, 184.0000000000000000, -7.000000000000000000 ) ) ;
#10533=VERTEX_POINT ( 'NONE', #990 ) ;
#10558=VERTEX_POINT ( 'NONE', #12047 ) ;
#10577=CARTESIAN_POINT ( 'NONE',  ( 4.000000000000002665, 184.0000000000000000, -7.000000000000000888 ) ) ;
#10587=EDGE_CURVE ( 'NONE', #2813, #8352, #10854, .T. ) ;
#10601=AXIS2_PLACEMENT_3D ( 'NONE', #2214, #6855, #1981 ) ;
#10612=CARTESIAN_POINT ( 'NONE',  ( 0.000000000000000000, 184.0000000000000000, 7.000000000000000000 ) ) ;
#10636=LINE ( 'NONE', #15256, #12469 ) ;
#10674=ORIENTED_EDGE ( 'NONE', *, *, #9620, .T. ) ;
#10717=ORIENTED_EDGE ( 'NONE', *, *, #6297, .T. ) ;
#10734=DIRECTION ( 'NONE',  ( -0.000000000000000000, 1.000000000000000000, -0.000000000000000000 ) ) ;
#10737=DIRECTION ( 'NONE',  ( 0.000000000000000000, 0.000000000000000000, 1.000000000000000000 ) ) ;
#10760=EDGE_CURVE ( 'NONE', #2054, #13232, #14995, .T. ) ;
#10805=EDGE_CURVE ( 'NONE', #8352, #260, #15392, .T. ) ;
#10854=LINE ( 'NONE', #15720, #11060 ) ;
#10945=ORIENTED_EDGE ( 'NONE', *, *, #4965, .T. ) ;
#10992=DIRECTION ( 'NONE',  ( 0.000000000000000000, 0.000000000000000000, -1.000000000000000000 ) ) ;
#10996=CARTESIAN_POINT ( 'NONE',  ( 0.000000000000000000, 184.0000000000000000, -7.000000000000000000 ) ) ;
#11038=DIRECTION ( 'NONE',  ( 0.000000000000000000, 0.000000000000000000, 1.000000000000000000 ) ) ;
#11049=FACE_OUTER_BOUND ( 'NONE', #8540, .T. ) ;
#11060=VECTOR ( 'NONE', #4820, 1000.000000000000000 ) ;
#11068=CARTESIAN_POINT ( 'NONE',  ( 0.000000000000000000, 182.0000000000000000, 0.000000000000000000 ) ) ;
#11100=VERTEX_POINT ( 'NONE', #7381 ) ;
#11110=SURFACE_STYLE_FILL_AREA ( #2279 ) ;
#11114=VECTOR ( 'NONE', #6775, 1000.000000000000000 ) ;
#11125=AXIS2_PLACEMENT_3D ( 'NONE', #2579, #5506, #4142 ) ;
#11193=DIRECTION ( 'NONE',  ( 1.000000000000000000, 0.000000000000000000, 0.000000000000000000 ) ) ;
#11195=DIRECTION ( 'NONE',  ( 1.000000000000000000, 0.000000000000000000, 0.000000000000000000 ) ) ;
#11198=FACE_OUTER_BOUND ( 'NONE', #9746, .T. ) ;
#11217=EDGE_LOOP ( 'NONE', ( #1019, #9403, #2324, #3487 ) ) ;
#11220=PLANE ( 'NONE',  #4793 ) ;
#11234=ORIENTED_EDGE ( 'NONE', *, *, #9620, .F. ) ;
#11249=DIRECTION ( 'NONE',  ( 0.000000000000000000, 0.000000000000000000, -1.000000000000000000 ) ) ;
#11272=FACE_OUTER_BOUND ( 'NONE', #5361, .T. ) ;
#11299=CARTESIAN_POINT ( 'NONE',  ( 0.000000000000000000, 182.0000000000000000, 0.000000000000000000 ) ) ;
#11337=DIRECTION ( 'NONE',  ( -0.000000000000000000, 1.000000000000000000, -0.000000000000000000 ) ) ;
#11373=ORIENTED_EDGE ( 'NONE', *, *, #3786, .F. ) ;
#11391=CIRCLE ( 'NONE', #14179, 4.000000000000001776 ) ;
#11393=MECHANICAL_DESIGN_GEOMETRIC_PRESENTATION_REPRESENTATION('',(#8367),#13683);
#11426=DIRECTION ( 'NONE',  ( 0.000000000000000000, 0.000000000000000000, 1.000000000000000000 ) ) ;
#11453=ORIENTED_EDGE ( 'NONE', *, *, #13975, .F. ) ;
#11459=FACE_BOUND ( 'NONE', #3175, .T. ) ;
#11476=DIRECTION ( 'NONE',  ( -0.000000000000000000, 1.000000000000000000, -0.000000000000000000 ) ) ;
#11486=ORIENTED_EDGE ( 'NONE', *, *, #2984, .F. ) ;
#11496=CARTESIAN_POINT ( 'NONE',  ( 0.000000000000000000, 184.0000000000000000, -7.000000000000000000 ) ) ;
#11513=DIRECTION ( 'NONE',  ( 0.000000000000000000, 0.000000000000000000, 1.000000000000000000 ) ) ;
#11630=EDGE_CURVE ( 'NONE', #14401, #14543, #14080, .T. ) ;
#11844=PLANE ( 'NONE',  #7703 ) ;
#11849=CARTESIAN_POINT ( 'NONE',  ( 0.000000000000000000, 182.0000000000000000, -3.000000000000000888 ) ) ;
#11877=UNCERTAINTY_MEASURE_WITH_UNIT (LENGTH_MEASURE( 1.000000000000000082E-05 ), #13761, 'distance_accuracy_value', 'NONE');
#11955=EDGE_LOOP ( 'NONE', ( #11453, #622, #14961, #8419 ) ) ;
#12008=CARTESIAN_POINT ( 'NONE',  ( 0.000000000000000000, 184.0000000000000000, -3.000000000000000888 ) ) ;
#12017=ORIENTED_EDGE ( 'NONE', *, *, #4055, .F. ) ;
#12031=DIRECTION ( 'NONE',  ( 0.000000000000000000, 0.000000000000000000, 1.000000000000000000 ) ) ;
#12039=CIRCLE ( 'NONE', #3901, 4.000000000000002665 ) ;
#12047=CARTESIAN_POINT ( 'NONE',  ( 0.000000000000000000, 182.0000000000000000, -12.49999999999999822 ) ) ;
#12092=EDGE_CURVE ( 'NONE', #6866, #1061, #8004, .T. ) ;
#12132=PRODUCT_DEFINITION_FORMATION_WITH_SPECIFIED_SOURCE ( 'ANY', '', #166, .NOT_KNOWN. ) ;
#12135=VERTEX_POINT ( 'NONE', #3478 ) ;
#12193=VERTEX_POINT ( 'NONE', #2682 ) ;
#12213=DIRECTION ( 'NONE',  ( -0.000000000000000000, 1.000000000000000000, -0.000000000000000000 ) ) ;
#12227=CARTESIAN_POINT ( 'NONE',  ( 9.750000000000003553, 184.0000000000000000, 1.020968533498575461E-13 ) ) ;
#12250=EDGE_CURVE ( 'NONE', #8636, #12288, #5530, .T. ) ;
#12255=FACE_BOUND ( 'NONE', #640, .T. ) ;
#12262=DIRECTION ( 'NONE',  ( -1.000000000000000000, 0.000000000000000000, 0.000000000000000000 ) ) ;
#12271=ADVANCED_FACE ( 'NONE', ( #10456 ), #1931, .F. ) ;
#12276=AXIS2_PLACEMENT_3D ( 'NONE', #5430, #14817, #13608 ) ;
#12281=DIRECTION ( 'NONE',  ( 0.000000000000000000, -1.000000000000000000, 0.000000000000000000 ) ) ;
#12288=VERTEX_POINT ( 'NONE', #6805 ) ;
#12294=DIRECTION ( 'NONE',  ( -6.123233995736766036E-17, 1.000000000000000000, 0.000000000000000000 ) ) ;
#12313=AXIS2_PLACEMENT_3D ( 'NONE', #14215, #4444, #12863 ) ;
#12380=ADVANCED_BREP_SHAPE_REPRESENTATION ( '', ( #4943, #14201 ), #4042 ) ;
#12408=EDGE_LOOP ( 'NONE', ( #4549, #3718 ) ) ;
#12411=DIRECTION ( 'NONE',  ( 0.000000000000000000, -0.000000000000000000, -1.000000000000000000 ) ) ;
#12469=VECTOR ( 'NONE', #6988, 1000.000000000000000 ) ;
#12473=CYLINDRICAL_SURFACE ( 'NONE', #999, 2.499999999999999556 ) ;
#12481=CARTESIAN_POINT ( 'NONE',  ( -3.061616997868391523E-16, 189.0000000000000000, -4.500000000000000888 ) ) ;
#12495=CARTESIAN_POINT ( 'NONE',  ( 0.000000000000000000, 184.0000000000000000, -12.49999999999999822 ) ) ;
#12516=CIRCLE ( 'NONE', #8472, 3.000000000000000888 ) ;
#12531=CARTESIAN_POINT ( 'NONE',  ( 9.750000000000003553, 184.0000000000000000, -1.499999999999897415 ) ) ;
#12534=CARTESIAN_POINT ( 'NONE',  ( 9.750000000000003553, 182.0000000000000000, 1.500000000000101696 ) ) ;
#12540=CARTESIAN_POINT ( 'NONE',  ( -3.061616997868386099E-16, 189.0000000000000000, 7.000000000000000000 ) ) ;
#12555=DIRECTION ( 'NONE',  ( -0.000000000000000000, 1.000000000000000000, -0.000000000000000000 ) ) ;
#12567=DIRECTION ( 'NONE',  ( 0.000000000000000000, 0.000000000000000000, 1.000000000000000000 ) ) ;
#12574=DIRECTION ( 'NONE',  ( 0.000000000000000000, 0.000000000000000000, -1.000000000000000000 ) ) ;
#12586=ORIENTED_EDGE ( 'NONE', *, *, #1912, .T. ) ;
#12608=AXIS2_PLACEMENT_3D ( 'NONE', #1347, #3735, #8612 ) ;
#12635=CARTESIAN_POINT ( 'NONE',  ( -9.750000000000003553, 182.0000000000000000, -1.500000000000033751 ) ) ;
#12645=CARTESIAN_POINT ( 'NONE',  ( 0.000000000000000000, 184.0000000000000000, 0.000000000000000000 ) ) ;
#12649=ADVANCED_FACE ( 'NONE', ( #11198 ), #5242, .F. ) ;
#12663=AXIS2_PLACEMENT_3D ( 'NONE', #1388, #6263, #7600 ) ;
#12750=EDGE_CURVE ( 'NONE', #1061, #9576, #2110, .T. ) ;
#12837=EDGE_LOOP ( 'NONE', ( #7409, #7488 ) ) ;
#12848=FACE_OUTER_BOUND ( 'NONE', #7485, .T. ) ;
#12863=DIRECTION ( 'NONE',  ( 0.000000000000000000, 0.000000000000000000, 1.000000000000000000 ) ) ;
#12950=VERTEX_POINT ( 'NONE', #896 ) ;
#12972=ADVANCED_FACE ( 'NONE', ( #12985 ), #700, .T. ) ;
#12985=FACE_OUTER_BOUND ( 'NONE', #7700, .T. ) ;
#13010=AXIS2_PLACEMENT_3D ( 'NONE', #11496, #14040, #7765 ) ;
#13036=CARTESIAN_POINT ( 'NONE',  ( -3.061616997868391523E-16, 189.0000000000000000, -7.000000000000000000 ) ) ;
#13063=DIRECTION ( 'NONE',  ( 0.000000000000000000, 0.000000000000000000, 1.000000000000000000 ) ) ;
#13086=CARTESIAN_POINT ( 'NONE',  ( -9.750000000000003553, 184.0000000000000000, -1.500000000000033751 ) ) ;
#13088=LINE ( 'NONE', #6107, #6832 ) ;
#13148=ORIENTED_EDGE ( 'NONE', *, *, #13975, .T. ) ;
#13180=FILL_AREA_STYLE_COLOUR ( '', #6092 ) ;
#13201=FACE_BOUND ( 'NONE', #14527, .T. ) ;
#13212=ORIENTED_EDGE ( 'NONE', *, *, #4476, .F. ) ;
#13232=VERTEX_POINT ( 'NONE', #4610 ) ;
#13254=DIRECTION ( 'NONE',  ( 0.000000000000000000, -1.000000000000000000, 0.000000000000000000 ) ) ;
#13327=EDGE_CURVE ( 'NONE', #10284, #9576, #10118, .T. ) ;
#13351=VECTOR ( 'NONE', #11476, 1000.000000000000000 ) ;
#13362=CARTESIAN_POINT ( 'NONE',  ( 9.750000000000003553, 184.0000000000000000, 1.500000000000101696 ) ) ;
#13391=AXIS2_PLACEMENT_3D ( 'NONE', #12540, #6357, #11193 ) ;
#13419=SURFACE_STYLE_USAGE ( .BOTH. , #215 ) ;
#13437=CARTESIAN_POINT ( 'NONE',  ( -9.148167235839370302E-31, 182.0000000000000000, 4.500000000000000888 ) ) ;
#13452=ORIENTED_EDGE ( 'NONE', *, *, #3504, .F. ) ;
#13453=FACE_OUTER_BOUND ( 'NONE', #14507, .T. ) ;
#13454=EDGE_LOOP ( 'NONE', ( #9121, #4311, #6067, #8946 ) ) ;
#13468=ORIENTED_EDGE ( 'NONE', *, *, #3370, .T. ) ;
#13502=DIRECTION ( 'NONE',  ( -0.000000000000000000, 1.000000000000000000, -0.000000000000000000 ) ) ;
#13545=CARTESIAN_POINT ( 'NONE',  ( -3.118365096457675456, 189.0000000000000000, -7.000000000000000000 ) ) ;
#13602=ORIENTED_EDGE ( 'NONE', *, *, #13327, .T. ) ;
#13608=DIRECTION ( 'NONE',  ( 0.000000000000000000, -0.000000000000000000, -1.000000000000000000 ) ) ;
#13620=ORIENTED_EDGE ( 'NONE', *, *, #6297, .F. ) ;
#13659=AXIS2_PLACEMENT_3D ( 'NONE', #8609, #3732, #4781 ) ;
#13683=( GEOMETRIC_REPRESENTATION_CONTEXT ( 3 ) GLOBAL_UNCERTAINTY_ASSIGNED_CONTEXT ( ( #11877 ) ) GLOBAL_UNIT_ASSIGNED_CONTEXT ( ( #13761, #8849, #6696 ) ) REPRESENTATION_CONTEXT ( 'NONE', 'WORKASPACE' ) );
#13716=EDGE_CURVE ( 'NONE', #6866, #10284, #13088, .T. ) ;
#13761=( LENGTH_UNIT ( ) NAMED_UNIT ( * ) SI_UNIT ( .MILLI., .METRE. ) );
#13819=DIRECTION ( 'NONE',  ( 1.000000000000000000, 0.000000000000000000, 0.000000000000000000 ) ) ;
#13828=DIRECTION ( 'NONE',  ( -0.000000000000000000, 1.000000000000000000, -0.000000000000000000 ) ) ;
#13844=FACE_BOUND ( 'NONE', #12408, .T. ) ;
#13893=VERTEX_POINT ( 'NONE', #1701 ) ;
#13897=AXIS2_PLACEMENT_3D ( 'NONE', #4859, #7245, #4777 ) ;
#13899=CARTESIAN_POINT ( 'NONE',  ( -3.061616997868391523E-16, 189.0000000000000000, 7.000000000000000000 ) ) ;
#13916=CARTESIAN_POINT ( 'NONE',  ( 0.000000000000000000, 184.0000000000000000, 7.000000000000000000 ) ) ;
#13927=EDGE_LOOP ( 'NONE', ( #15060, #6535, #5745, #7832 ) ) ;
#13959=CYLINDRICAL_SURFACE ( 'NONE', #2071, 2.499999999999999556 ) ;
#13975=EDGE_CURVE ( 'NONE', #2054, #11100, #8866, .T. ) ;
#13992=CARTESIAN_POINT ( 'NONE',  ( -9.750000000000003553, 184.0000000000000000, -3.401296724241641415E-14 ) ) ;
#13993=VERTEX_POINT ( 'NONE', #2670 ) ;
#14001=DIRECTION ( 'NONE',  ( -0.000000000000000000, 1.000000000000000000, -0.000000000000000000 ) ) ;
#14028=CARTESIAN_POINT ( 'NONE',  ( -8.666684749742561339E-31, 189.0000000000000000, -9.500000000000000000 ) ) ;
#14034=CIRCLE ( 'NONE', #5421, 3.000000000000000888 ) ;
#14040=DIRECTION ( 'NONE',  ( -6.123233995736766036E-17, 1.000000000000000000, 0.000000000000000000 ) ) ;
#14055=( LENGTH_UNIT ( ) NAMED_UNIT ( * ) SI_UNIT ( .MILLI., .METRE. ) );
#14062=DIRECTION ( 'NONE',  ( -1.000000000000000000, 0.000000000000000000, 0.000000000000000000 ) ) ;
#14071=FACE_OUTER_BOUND ( 'NONE', #4230, .T. ) ;
#14079=DIRECTION ( 'NONE',  ( 6.123233995736766036E-17, -1.000000000000000000, -0.000000000000000000 ) ) ;
#14080=CIRCLE ( 'NONE', #3672, 3.000000000000000888 ) ;
#14129=EDGE_CURVE ( 'NONE', #260, #10533, #11391, .T. ) ;
#14159=CIRCLE ( 'NONE', #2484, 4.000000000000001776 ) ;
#14161=ORIENTED_EDGE ( 'NONE', *, *, #12092, .F. ) ;
#14179=AXIS2_PLACEMENT_3D ( 'NONE', #10612, #4812, #6003 ) ;
#14198=DIRECTION ( 'NONE',  ( -0.000000000000000000, 1.000000000000000000, -0.000000000000000000 ) ) ;
#14201=AXIS2_PLACEMENT_3D ( 'NONE', #6680, #11513, #1651 ) ;
#14215=CARTESIAN_POINT ( 'NONE',  ( -9.750000000000003553, 182.0000000000000000, -3.401296724241641415E-14 ) ) ;
#14222=VERTEX_POINT ( 'NONE', #13545 ) ;
#14284=CONICAL_SURFACE ( 'NONE', #2615, 4.000000000000002665, 0.1745329251994333364 ) ;
#14332=DIRECTION ( 'NONE',  ( 1.000000000000000000, 0.000000000000000000, 0.000000000000000000 ) ) ;
#14401=VERTEX_POINT ( 'NONE', #6791 ) ;
#14411=VECTOR ( 'NONE', #7126, 1000.000000000000000 ) ;
#14429=UNCERTAINTY_MEASURE_WITH_UNIT (LENGTH_MEASURE( 1.000000000000000082E-05 ), #6034, 'distance_accuracy_value', 'NONE');
#14448=COLOUR_RGB ( '', 0.66274510, 0.83137255, 0.94901961) ;
#14462=CIRCLE ( 'NONE', #6605, 2.499999999999999556 ) ;
#14503=ORIENTED_EDGE ( 'NONE', *, *, #5497, .T. ) ;
#14507=EDGE_LOOP ( 'NONE', ( #7864, #4229 ) ) ;
#14523=EDGE_LOOP ( 'NONE', ( #1833, #3889 ) ) ;
#14527=EDGE_LOOP ( 'NONE', ( #10205, #12017 ) ) ;
#14541=CIRCLE ( 'NONE', #8717, 2.499999999999999556 ) ;
#14543=VERTEX_POINT ( 'NONE', #11849 ) ;
#14552=FACE_OUTER_BOUND ( 'NONE', #15003, .T. ) ;
#14560=DIRECTION ( 'NONE',  ( -0.000000000000000000, 1.000000000000000000, -0.000000000000000000 ) ) ;
#14576=CARTESIAN_POINT ( 'NONE',  ( 3.673940397442060854E-16, 184.0000000000000000, 3.000000000000000888 ) ) ;
#14579=ADVANCED_FACE ( 'NONE', ( #7413, #14810, #2791, #12255, #14653, #13453 ), #11220, .T. ) ;
#14580=DIRECTION ( 'NONE',  ( -0.000000000000000000, 1.000000000000000000, -0.000000000000000000 ) ) ;
#14585=ORIENTED_EDGE ( 'NONE', *, *, #7801, .T. ) ;
#14618=VECTOR ( 'NONE', #182, 1000.000000000000000 ) ;
#14620=DIRECTION ( 'NONE',  ( -0.000000000000000000, 1.000000000000000000, -0.000000000000000000 ) ) ;
#14651=ORIENTED_EDGE ( 'NONE', *, *, #8176, .T. ) ;
#14653=FACE_BOUND ( 'NONE', #3974, .T. ) ;
#14667=ADVANCED_FACE ( 'NONE', ( #6539 ), #1743, .F. ) ;
#14698=PRESENTATION_STYLE_ASSIGNMENT (( #13419 ) ) ;
#14712=CIRCLE ( 'NONE', #6836, 2.499999999999999556 ) ;
#14770=EDGE_CURVE ( 'NONE', #13893, #14222, #3523, .T. ) ;
#14789=EDGE_LOOP ( 'NONE', ( #11486, #2254 ) ) ;
#14797=CIRCLE ( 'NONE', #803, 3.118365096457675012 ) ;
#14810=FACE_BOUND ( 'NONE', #12837, .T. ) ;
#14811=ORIENTED_EDGE ( 'NONE', *, *, #842, .T. ) ;
#14817=DIRECTION ( 'NONE',  ( 0.000000000000000000, -1.000000000000000000, 0.000000000000000000 ) ) ;
#14846=CARTESIAN_POINT ( 'NONE',  ( -9.750000000000003553, 184.0000000000000000, -3.401296724241641415E-14 ) ) ;
#14863=ADVANCED_FACE ( 'NONE', ( #2948 ), #7796, .F. ) ;
#14877=CIRCLE ( 'NONE', #8790, 1.499999999999999556 ) ;
#14878=EDGE_LOOP ( 'NONE', ( #11373, #9118 ) ) ;
#14930=ADVANCED_FACE ( 'NONE', ( #3010 ), #12473, .F. ) ;
#14945=AXIS2_PLACEMENT_3D ( 'NONE', #7724, #12281, #12574 ) ;
#14961=ORIENTED_EDGE ( 'NONE', *, *, #7655, .T. ) ;
#14981=ORIENTED_EDGE ( 'NONE', *, *, #14770, .F. ) ;
#14988=ORIENTED_EDGE ( 'NONE', *, *, #2105, .F. ) ;
#14995=LINE ( 'NONE', #650, #13351 ) ;
#15003=EDGE_LOOP ( 'NONE', ( #10717, #658 ) ) ;
#15034=DIRECTION ( 'NONE',  ( 0.000000000000000000, -1.000000000000000000, 0.000000000000000000 ) ) ;
#15060=ORIENTED_EDGE ( 'NONE', *, *, #8486, .F. ) ;
#15079=ORIENTED_EDGE ( 'NONE', *, *, #3402, .T. ) ;
#15163=CARTESIAN_POINT ( 'NONE',  ( -3.061616997868391523E-16, 189.0000000000000000, 7.000000000000000000 ) ) ;
#15197=CIRCLE ( 'NONE', #13659, 12.49999999999999822 ) ;
#15256=CARTESIAN_POINT ( 'NONE',  ( -3.061616997868391523E-16, 189.0000000000000000, 9.500000000000000000 ) ) ;
#15308=DIRECTION ( 'NONE',  ( -0.000000000000000000, 1.000000000000000000, -0.000000000000000000 ) ) ;
#15382=PRODUCT_CONTEXT ( 'NONE', #5877, 'mechanical' ) ;
#15392=CIRCLE ( 'NONE', #4200, 4.000000000000001776 ) ;
#15397=ORIENTED_EDGE ( 'NONE', *, *, #4965, .F. ) ;
#15411=CIRCLE ( 'NONE', #4231, 1.499999999999999556 ) ;
#15446=CARTESIAN_POINT ( 'NONE',  ( -3.061616997868383141E-16, 189.0000000000000000, 7.000000000000000000 ) ) ;
#15465=DIRECTION ( 'NONE',  ( -0.000000000000000000, 1.000000000000000000, -0.000000000000000000 ) ) ;
#15511=DIRECTION ( 'NONE',  ( -0.000000000000000000, 1.000000000000000000, -0.000000000000000000 ) ) ;
#15514=ADVANCED_FACE ( 'NONE', ( #9177 ), #9029, .F. ) ;
#15548=CARTESIAN_POINT ( 'NONE',  ( 0.000000000000000000, 184.0000000000000000, 7.000000000000000000 ) ) ;
#15554=ORIENTED_EDGE ( 'NONE', *, *, #10587, .T. ) ;
#15604=VECTOR ( 'NONE', #1658, 1000.000000000000000 ) ;
#15698=CARTESIAN_POINT ( 'NONE',  ( -8.185202263645752375E-31, 182.0000000000000000, -9.500000000000000000 ) ) ;
#15707=AXIS2_PLACEMENT_3D ( 'NONE', #15548, #2247, #14332 ) ;
#15720=CARTESIAN_POINT ( 'NONE',  ( -4.000000000000001776, 184.0000000000000000, 7.000000000000000888 ) ) ;
ENDSEC;
END-ISO-10303-21;
